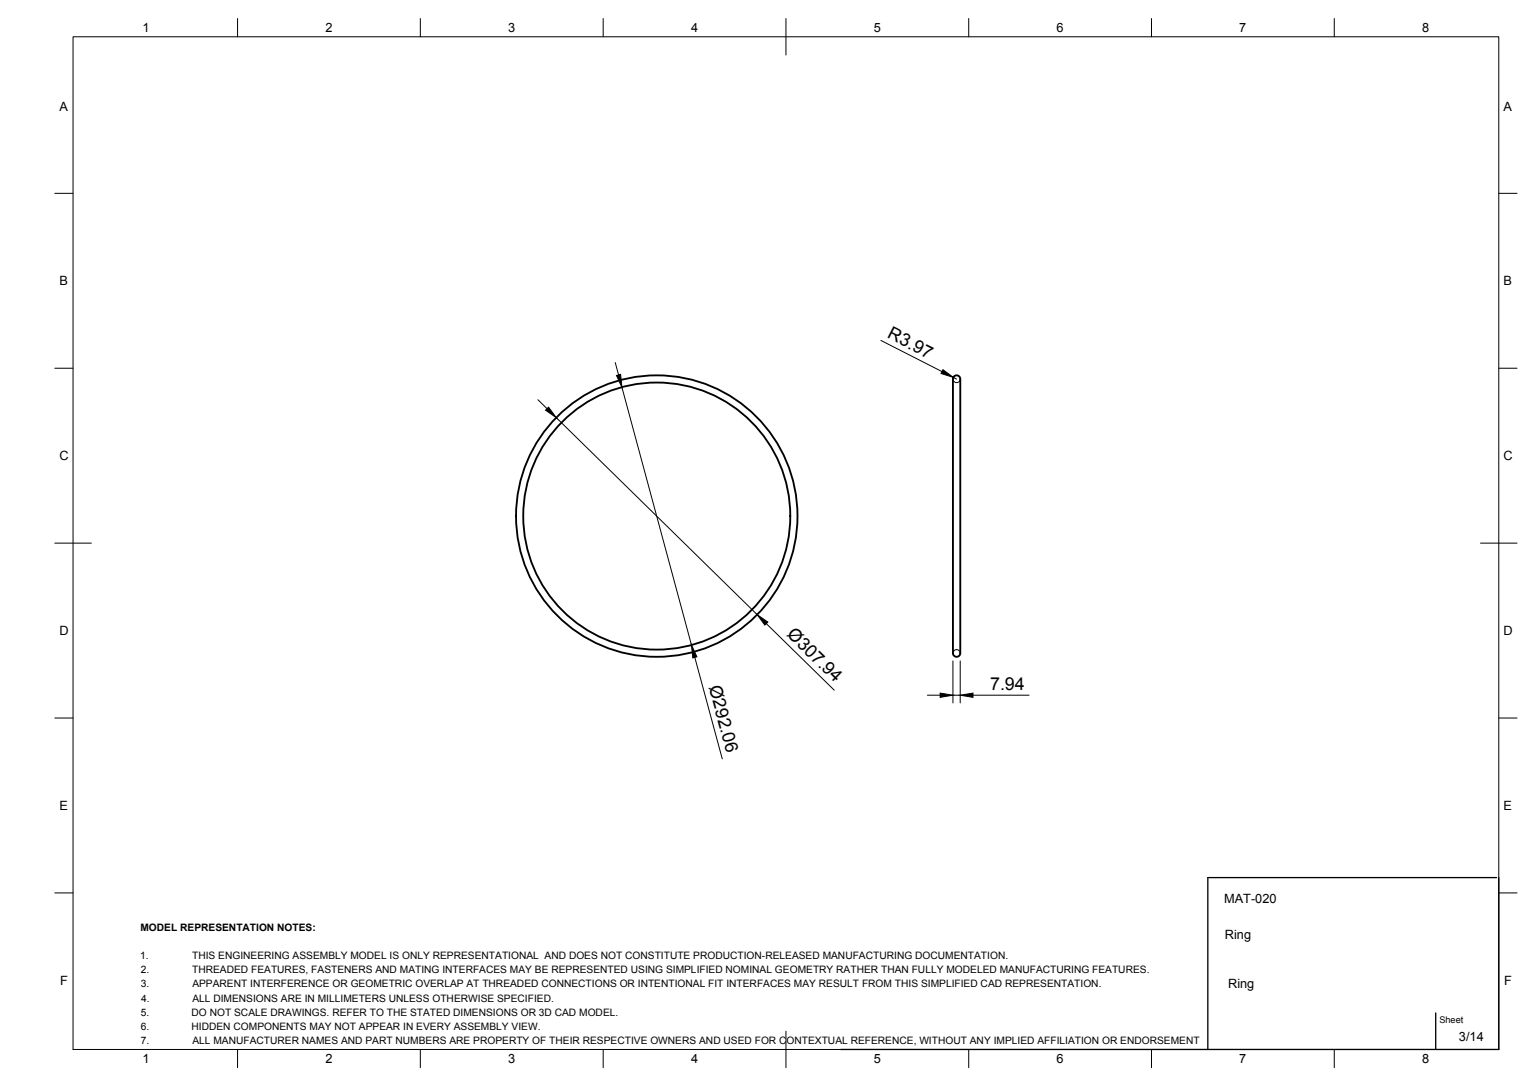
ISO-10303-21;
HEADER;
/* Generated by software containing ST-Developer
 * from STEP Tools, Inc. (www.steptools.com) 
 */

FILE_DESCRIPTION(
/* description */ ('STEP AP214'),
/* implementation_level */ '2;1');

FILE_NAME(
/* name */ 'Ring.step',
/* time_stamp */ '2026-11-14T06:20:50-08:00',
/* author */ (''),
/* organization */ (''),
/* preprocessor_version */ 'ST-DEVELOPER v20.2',
/* originating_system */ 'Autodesk Translation Framework v15.17.0.0',
/* authorisation */ '');

FILE_SCHEMA (('AUTOMOTIVE_DESIGN { 1 0 10303 214 3 1 1 }'));
ENDSEC;

DATA;
#10=MECHANICAL_DESIGN_GEOMETRIC_PRESENTATION_REPRESENTATION('',(#956),#20658);
#932=SHAPE_REPRESENTATION_RELATIONSHIP('SRR','None',#20716,#944);
#944=ADVANCED_BREP_SHAPE_REPRESENTATION('',(#968),#20646);
#956=STYLED_ITEM('',(#20785),#968);
#968=MANIFOLD_SOLID_BREP('Body1',#3651);
#980=FACE_OUTER_BOUND('',#1189,.T.);
#1189=EDGE_LOOP('',(#2402,#2403,#2404,#2405));
#1421=CIRCLE('',#3799,3.96875);
#1422=CIRCLE('',#3800,146.03125);
#1546=VERTEX_POINT('',#4991);
#1883=EDGE_CURVE('',#1546,#1546,#1421,.T.);
#1884=EDGE_CURVE('',#1546,#1546,#1422,.T.);
#2402=ORIENTED_EDGE('',*,*,#1883,.F.);
#2403=ORIENTED_EDGE('',*,*,#1884,.T.);
#2404=ORIENTED_EDGE('',*,*,#1883,.T.);
#2405=ORIENTED_EDGE('',*,*,#1884,.F.);
#3440=TOROIDAL_SURFACE('',#3798,150.,3.96875);
#3442=ADVANCED_FACE('',(#980),#3440,.T.);
#3651=CLOSED_SHELL('',(#3442));
#3797=AXIS2_PLACEMENT_3D('',#4989,#4131,#4132);
#3798=AXIS2_PLACEMENT_3D('',#4990,#4133,#4134);
#3799=AXIS2_PLACEMENT_3D('',#4992,#4135,#4136);
#3800=AXIS2_PLACEMENT_3D('',#4993,#4137,#4138);
#4131=DIRECTION('axis',(0.,0.,1.));
#4132=DIRECTION('refdir',(1.,0.,0.));
#4133=DIRECTION('center_axis',(0.,1.,0.));
#4134=DIRECTION('ref_axis',(0.,0.,1.));
#4135=DIRECTION('center_axis',(-1.,0.,1.15371258089726E-16));
#4136=DIRECTION('ref_axis',(-1.15371258089726E-16,0.,-1.));
#4137=DIRECTION('center_axis',(0.,-1.,0.));
#4138=DIRECTION('ref_axis',(0.,0.,1.));
#4989=CARTESIAN_POINT('',(0.,0.,0.));
#4990=CARTESIAN_POINT('Origin',(150.,0.,0.));
#4991=CARTESIAN_POINT('',(150.,4.86031698411606E-16,-146.03125));
#4992=CARTESIAN_POINT('Origin',(150.,0.,-150.));
#4993=CARTESIAN_POINT('Origin',(150.,-4.86031698411606E-16,0.));
#20632=UNCERTAINTY_MEASURE_WITH_UNIT(LENGTH_MEASURE(0.01),#20659,
'DISTANCE_ACCURACY_VALUE',
'Maximum model space distance between geometric entities at asserted c
onnectivities');
#20644=UNCERTAINTY_MEASURE_WITH_UNIT(LENGTH_MEASURE(0.01),#20659,
'DISTANCE_ACCURACY_VALUE',
'Maximum model space distance between geometric entities at asserted c
onnectivities');
#20646=(
GEOMETRIC_REPRESENTATION_CONTEXT(3)
GLOBAL_UNCERTAINTY_ASSIGNED_CONTEXT((#20632))
GLOBAL_UNIT_ASSIGNED_CONTEXT((#20659,#20661,#20662))
REPRESENTATION_CONTEXT('','3D')
);
#20658=(
GEOMETRIC_REPRESENTATION_CONTEXT(3)
GLOBAL_UNCERTAINTY_ASSIGNED_CONTEXT((#20644))
GLOBAL_UNIT_ASSIGNED_CONTEXT((#20659,#20661,#20662))
REPRESENTATION_CONTEXT('','3D')
);
#20659=(
LENGTH_UNIT()
NAMED_UNIT(*)
SI_UNIT(.MILLI.,.METRE.)
);
#20661=(
NAMED_UNIT(*)
PLANE_ANGLE_UNIT()
SI_UNIT($,.RADIAN.)
);
#20662=(
NAMED_UNIT(*)
SI_UNIT($,.STERADIAN.)
SOLID_ANGLE_UNIT()
);
#20664=SHAPE_DEFINITION_REPRESENTATION(#20677,#20716);
#20677=PRODUCT_DEFINITION_SHAPE('',$,#20730);
#20716=SHAPE_REPRESENTATION('',(#3797),#20646);
#20728=PRODUCT_DEFINITION_CONTEXT('part definition',#20769,'design');
#20730=PRODUCT_DEFINITION('Ring','Ring',#20743,#20728);
#20743=PRODUCT_DEFINITION_FORMATION('',$,#20772);
#20769=APPLICATION_CONTEXT(
'Core Data for Automotive Mechanical Design Process');
#20770=PRODUCT_CONTEXT('part definition',#20769,'mechanical');
#20772=PRODUCT('Ring','Ring',$,(#20770));
#20785=PRESENTATION_STYLE_ASSIGNMENT((#20790));
#20790=SURFACE_STYLE_USAGE(.BOTH.,#20795);
#20795=SURFACE_SIDE_STYLE('',(#20800));
#20800=SURFACE_STYLE_FILL_AREA(#20805);
#20805=FILL_AREA_STYLE('Opaque(97,158,199)',(#20810));
#20810=FILL_AREA_STYLE_COLOUR('Opaque(97,158,199)',#20815);
#20815=COLOUR_RGB('Opaque(97,158,199)',0.380392156862745,0.619607843137255,
0.780392156862745);
ENDSEC;
END-ISO-10303-21;
